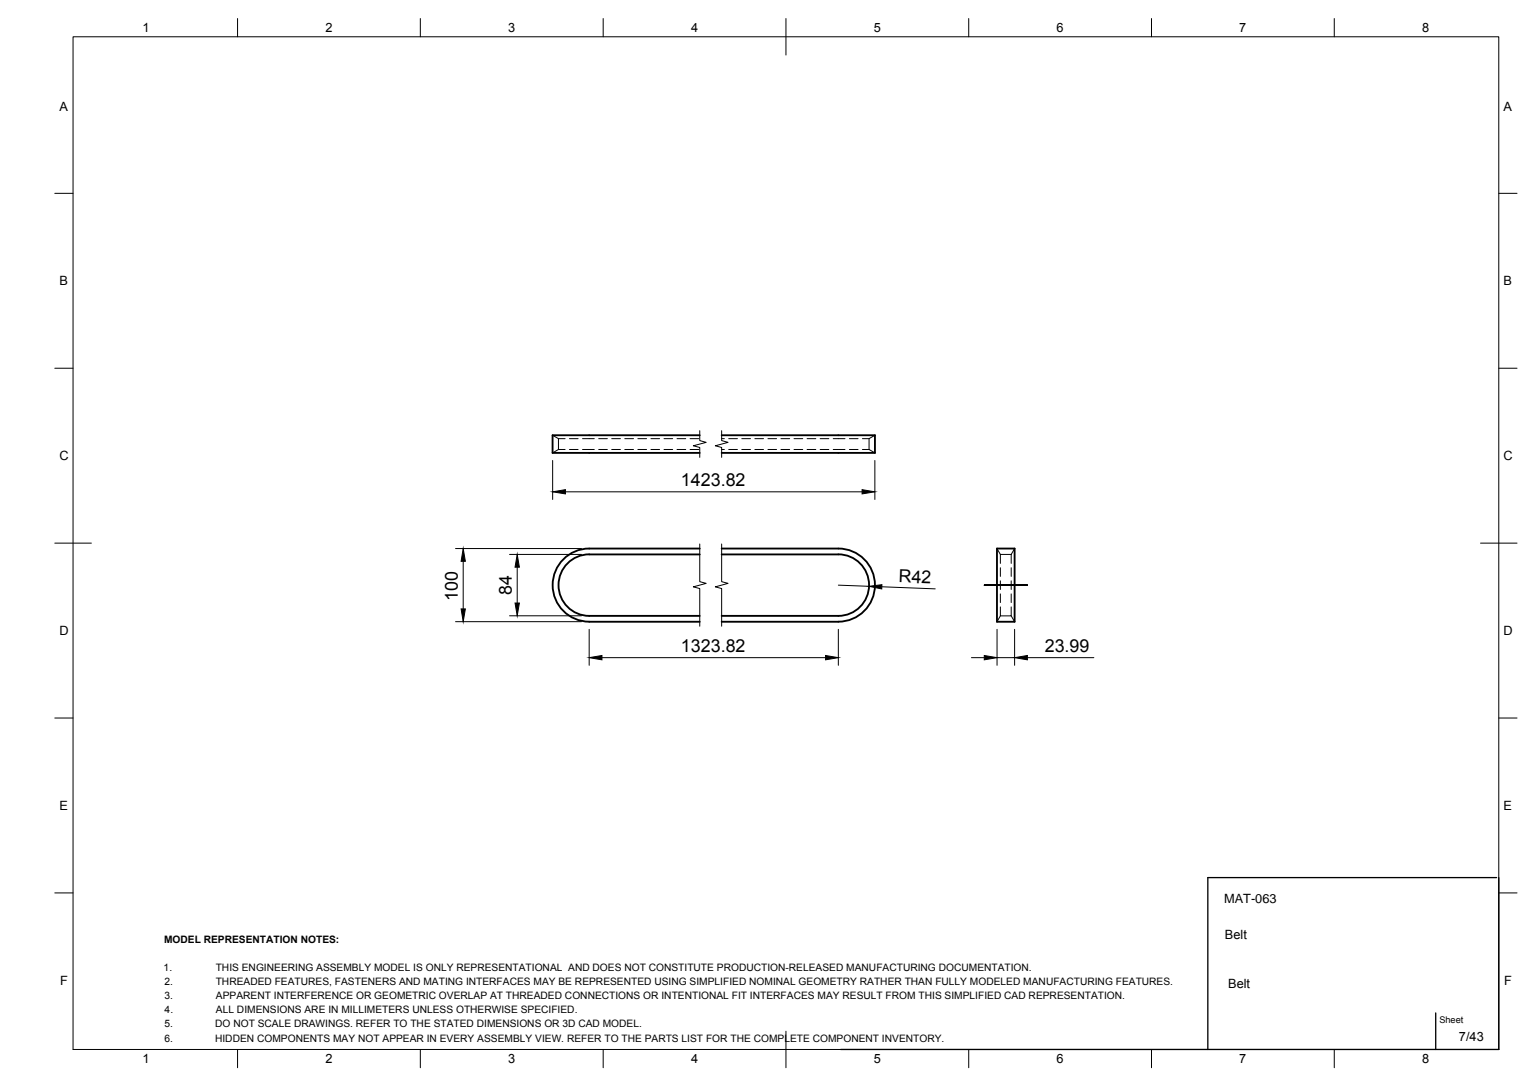
ISO-10303-21;
HEADER;
/* Generated by software containing ST-Developer
 * from STEP Tools, Inc. (www.steptools.com) 
 */

FILE_DESCRIPTION(
/* description */ (''),
/* implementation_level */ '2;1');

FILE_NAME(
/* name */ 'Belt.step',
/* time_stamp */ '2026-10-24T09:43:01-07:00',
/* author */ (''),
/* organization */ (''),
/* preprocessor_version */ 'ST-DEVELOPER v20.2',
/* originating_system */ 'Autodesk Translation Framework v15.15.0.0',
/* authorisation */ '');

FILE_SCHEMA (('AUTOMOTIVE_DESIGN { 1 0 10303 214 3 1 1 }'));
ENDSEC;

DATA;
#10=MECHANICAL_DESIGN_GEOMETRIC_PRESENTATION_REPRESENTATION('',(#277),#11112);
#211=SHAPE_REPRESENTATION_RELATIONSHIP('SRR','None',#11234,#244);
#244=ADVANCED_BREP_SHAPE_REPRESENTATION('',(#310),#11079);
#277=STYLED_ITEM('',(#11426),#310);
#310=MANIFOLD_SOLID_BREP('Belt',#6014);
#516=PLANE('',#6636);
#517=PLANE('',#6641);
#518=PLANE('',#6645);
#519=PLANE('',#6647);
#520=PLANE('',#6648);
#521=PLANE('',#6649);
#522=PLANE('',#6654);
#523=PLANE('',#6655);
#669=CONICAL_SURFACE('',#6637,1.,1.04719756558882);
#670=CONICAL_SURFACE('',#6639,1.,1.04719756558882);
#671=CONICAL_SURFACE('',#6650,1.,1.04719756558882);
#672=CONICAL_SURFACE('',#6652,1.,1.04719756558882);
#757=FACE_OUTER_BOUND('',#1165,.T.);
#758=FACE_OUTER_BOUND('',#1166,.T.);
#759=FACE_OUTER_BOUND('',#1167,.T.);
#760=FACE_OUTER_BOUND('',#1168,.T.);
#761=FACE_OUTER_BOUND('',#1169,.T.);
#762=FACE_OUTER_BOUND('',#1170,.T.);
#763=FACE_OUTER_BOUND('',#1171,.T.);
#764=FACE_OUTER_BOUND('',#1172,.T.);
#765=FACE_OUTER_BOUND('',#1173,.T.);
#766=FACE_OUTER_BOUND('',#1174,.T.);
#767=FACE_OUTER_BOUND('',#1175,.T.);
#768=FACE_OUTER_BOUND('',#1176,.T.);
#769=FACE_OUTER_BOUND('',#1177,.T.);
#770=FACE_OUTER_BOUND('',#1178,.T.);
#771=FACE_OUTER_BOUND('',#1179,.T.);
#772=FACE_OUTER_BOUND('',#1180,.T.);
#1165=EDGE_LOOP('',(#4313,#4314,#4315,#4316));
#1166=EDGE_LOOP('',(#4317,#4318,#4319,#4320));
#1167=EDGE_LOOP('',(#4321,#4322,#4323,#4324));
#1168=EDGE_LOOP('',(#4325,#4326,#4327,#4328));
#1169=EDGE_LOOP('',(#4329,#4330,#4331,#4332));
#1170=EDGE_LOOP('',(#4333,#4334,#4335,#4336));
#1171=EDGE_LOOP('',(#4337,#4338,#4339,#4340));
#1172=EDGE_LOOP('',(#4341,#4342,#4343,#4344));
#1173=EDGE_LOOP('',(#4345,#4346,#4347,#4348));
#1174=EDGE_LOOP('',(#4349,#4350,#4351,#4352));
#1175=EDGE_LOOP('',(#4353,#4354,#4355,#4356));
#1176=EDGE_LOOP('',(#4357,#4358,#4359,#4360));
#1177=EDGE_LOOP('',(#4361,#4362,#4363,#4364));
#1178=EDGE_LOOP('',(#4365,#4366,#4367,#4368));
#1179=EDGE_LOOP('',(#4369,#4370,#4371,#4372));
#1180=EDGE_LOOP('',(#4373,#4374,#4375,#4376));
#1602=LINE('',#9716,#1961);
#1603=LINE('',#9719,#1962);
#1604=LINE('',#9722,#1963);
#1605=LINE('',#9724,#1964);
#1606=LINE('',#9725,#1965);
#1607=LINE('',#9728,#1966);
#1608=LINE('',#9731,#1967);
#1609=LINE('',#9736,#1968);
#1610=LINE('',#9737,#1969);
#1611=LINE('',#9740,#1970);
#1612=LINE('',#9741,#1971);
#1613=LINE('',#9745,#1972);
#1614=LINE('',#9750,#1973);
#1615=LINE('',#9751,#1974);
#1616=LINE('',#9753,#1975);
#1617=LINE('',#9754,#1976);
#1618=LINE('',#9756,#1977);
#1619=LINE('',#9757,#1978);
#1620=LINE('',#9760,#1979);
#1621=LINE('',#9761,#1980);
#1622=LINE('',#9763,#1981);
#1623=LINE('',#9767,#1982);
#1624=LINE('',#9771,#1983);
#1625=LINE('',#9773,#1984);
#1961=VECTOR('',#7760,0.01);
#1962=VECTOR('',#7763,0.01);
#1963=VECTOR('',#7766,0.01);
#1964=VECTOR('',#7767,0.01);
#1965=VECTOR('',#7768,0.01);
#1966=VECTOR('',#7771,0.01);
#1967=VECTOR('',#7774,0.01);
#1968=VECTOR('',#7779,0.01);
#1969=VECTOR('',#7780,0.01);
#1970=VECTOR('',#7783,0.01);
#1971=VECTOR('',#7784,0.01);
#1972=VECTOR('',#7787,0.01);
#1973=VECTOR('',#7794,0.01);
#1974=VECTOR('',#7795,0.01);
#1975=VECTOR('',#7798,0.01);
#1976=VECTOR('',#7799,0.01);
#1977=VECTOR('',#7802,0.01);
#1978=VECTOR('',#7803,0.01);
#1979=VECTOR('',#7806,0.01);
#1980=VECTOR('',#7807,0.01);
#1981=VECTOR('',#7810,0.01);
#1982=VECTOR('',#7815,0.01);
#1983=VECTOR('',#7822,0.01);
#1984=VECTOR('',#7825,0.01);
#2412=CIRCLE('',#6634,0.042);
#2413=CIRCLE('',#6635,0.042);
#2414=CIRCLE('',#6638,0.05);
#2415=CIRCLE('',#6640,0.05);
#2416=CIRCLE('',#6643,0.0419999999999999);
#2417=CIRCLE('',#6644,0.0420000000000001);
#2418=CIRCLE('',#6651,0.05);
#2419=CIRCLE('',#6653,0.0500000000000661);
#2798=VERTEX_POINT('',#9712);
#2799=VERTEX_POINT('',#9713);
#2800=VERTEX_POINT('',#9715);
#2801=VERTEX_POINT('',#9717);
#2802=VERTEX_POINT('',#9721);
#2803=VERTEX_POINT('',#9723);
#2804=VERTEX_POINT('',#9727);
#2805=VERTEX_POINT('',#9729);
#2806=VERTEX_POINT('',#9733);
#2807=VERTEX_POINT('',#9734);
#2808=VERTEX_POINT('',#9739);
#2809=VERTEX_POINT('',#9743);
#2810=VERTEX_POINT('',#9744);
#2811=VERTEX_POINT('',#9749);
#2812=VERTEX_POINT('',#9759);
#2813=VERTEX_POINT('',#9765);
#3360=EDGE_CURVE('',#2798,#2799,#2412,.F.);
#3361=EDGE_CURVE('',#2800,#2798,#1602,.F.);
#3362=EDGE_CURVE('',#2801,#2800,#2413,.F.);
#3363=EDGE_CURVE('',#2799,#2801,#1603,.F.);
#3364=EDGE_CURVE('',#2802,#2801,#1604,.T.);
#3365=EDGE_CURVE('',#2803,#2802,#1605,.T.);
#3366=EDGE_CURVE('',#2799,#2803,#1606,.T.);
#3367=EDGE_CURVE('',#2804,#2800,#1607,.F.);
#3368=EDGE_CURVE('',#2805,#2804,#2414,.F.);
#3369=EDGE_CURVE('',#2801,#2805,#1608,.F.);
#3370=EDGE_CURVE('',#2806,#2807,#2415,.F.);
#3371=EDGE_CURVE('',#2798,#2806,#1609,.F.);
#3372=EDGE_CURVE('',#2807,#2799,#1610,.F.);
#3373=EDGE_CURVE('',#2808,#2805,#1611,.T.);
#3374=EDGE_CURVE('',#2802,#2808,#1612,.T.);
#3375=EDGE_CURVE('',#2809,#2810,#1613,.F.);
#3376=EDGE_CURVE('',#2803,#2809,#2416,.F.);
#3377=EDGE_CURVE('',#2810,#2802,#2417,.F.);
#3378=EDGE_CURVE('',#2807,#2811,#1614,.T.);
#3379=EDGE_CURVE('',#2811,#2803,#1615,.T.);
#3380=EDGE_CURVE('',#2804,#2806,#1616,.F.);
#3381=EDGE_CURVE('',#2807,#2805,#1617,.F.);
#3382=EDGE_CURVE('',#2800,#2810,#1618,.T.);
#3383=EDGE_CURVE('',#2809,#2798,#1619,.T.);
#3384=EDGE_CURVE('',#2812,#2806,#1620,.T.);
#3385=EDGE_CURVE('',#2809,#2812,#1621,.T.);
#3386=EDGE_CURVE('',#2808,#2811,#1622,.T.);
#3387=EDGE_CURVE('',#2813,#2808,#2418,.F.);
#3388=EDGE_CURVE('',#2810,#2813,#1623,.F.);
#3389=EDGE_CURVE('',#2811,#2812,#2419,.F.);
#3390=EDGE_CURVE('',#2804,#2813,#1624,.T.);
#3391=EDGE_CURVE('',#2812,#2813,#1625,.T.);
#4313=ORIENTED_EDGE('',*,*,#3360,.F.);
#4314=ORIENTED_EDGE('',*,*,#3361,.F.);
#4315=ORIENTED_EDGE('',*,*,#3362,.F.);
#4316=ORIENTED_EDGE('',*,*,#3363,.F.);
#4317=ORIENTED_EDGE('',*,*,#3363,.T.);
#4318=ORIENTED_EDGE('',*,*,#3364,.F.);
#4319=ORIENTED_EDGE('',*,*,#3365,.F.);
#4320=ORIENTED_EDGE('',*,*,#3366,.F.);
#4321=ORIENTED_EDGE('',*,*,#3362,.T.);
#4322=ORIENTED_EDGE('',*,*,#3367,.F.);
#4323=ORIENTED_EDGE('',*,*,#3368,.F.);
#4324=ORIENTED_EDGE('',*,*,#3369,.F.);
#4325=ORIENTED_EDGE('',*,*,#3370,.F.);
#4326=ORIENTED_EDGE('',*,*,#3371,.F.);
#4327=ORIENTED_EDGE('',*,*,#3360,.T.);
#4328=ORIENTED_EDGE('',*,*,#3372,.F.);
#4329=ORIENTED_EDGE('',*,*,#3369,.T.);
#4330=ORIENTED_EDGE('',*,*,#3373,.F.);
#4331=ORIENTED_EDGE('',*,*,#3374,.F.);
#4332=ORIENTED_EDGE('',*,*,#3364,.T.);
#4333=ORIENTED_EDGE('',*,*,#3375,.F.);
#4334=ORIENTED_EDGE('',*,*,#3376,.F.);
#4335=ORIENTED_EDGE('',*,*,#3365,.T.);
#4336=ORIENTED_EDGE('',*,*,#3377,.F.);
#4337=ORIENTED_EDGE('',*,*,#3378,.F.);
#4338=ORIENTED_EDGE('',*,*,#3372,.T.);
#4339=ORIENTED_EDGE('',*,*,#3366,.T.);
#4340=ORIENTED_EDGE('',*,*,#3379,.F.);
#4341=ORIENTED_EDGE('',*,*,#3368,.T.);
#4342=ORIENTED_EDGE('',*,*,#3380,.T.);
#4343=ORIENTED_EDGE('',*,*,#3370,.T.);
#4344=ORIENTED_EDGE('',*,*,#3381,.T.);
#4345=ORIENTED_EDGE('',*,*,#3382,.F.);
#4346=ORIENTED_EDGE('',*,*,#3361,.T.);
#4347=ORIENTED_EDGE('',*,*,#3383,.F.);
#4348=ORIENTED_EDGE('',*,*,#3375,.T.);
#4349=ORIENTED_EDGE('',*,*,#3371,.T.);
#4350=ORIENTED_EDGE('',*,*,#3384,.F.);
#4351=ORIENTED_EDGE('',*,*,#3385,.F.);
#4352=ORIENTED_EDGE('',*,*,#3383,.T.);
#4353=ORIENTED_EDGE('',*,*,#3381,.F.);
#4354=ORIENTED_EDGE('',*,*,#3378,.T.);
#4355=ORIENTED_EDGE('',*,*,#3386,.F.);
#4356=ORIENTED_EDGE('',*,*,#3373,.T.);
#4357=ORIENTED_EDGE('',*,*,#3377,.T.);
#4358=ORIENTED_EDGE('',*,*,#3374,.T.);
#4359=ORIENTED_EDGE('',*,*,#3387,.F.);
#4360=ORIENTED_EDGE('',*,*,#3388,.F.);
#4361=ORIENTED_EDGE('',*,*,#3376,.T.);
#4362=ORIENTED_EDGE('',*,*,#3385,.T.);
#4363=ORIENTED_EDGE('',*,*,#3389,.F.);
#4364=ORIENTED_EDGE('',*,*,#3379,.T.);
#4365=ORIENTED_EDGE('',*,*,#3367,.T.);
#4366=ORIENTED_EDGE('',*,*,#3382,.T.);
#4367=ORIENTED_EDGE('',*,*,#3388,.T.);
#4368=ORIENTED_EDGE('',*,*,#3390,.F.);
#4369=ORIENTED_EDGE('',*,*,#3380,.F.);
#4370=ORIENTED_EDGE('',*,*,#3390,.T.);
#4371=ORIENTED_EDGE('',*,*,#3391,.F.);
#4372=ORIENTED_EDGE('',*,*,#3384,.T.);
#4373=ORIENTED_EDGE('',*,*,#3391,.T.);
#4374=ORIENTED_EDGE('',*,*,#3387,.T.);
#4375=ORIENTED_EDGE('',*,*,#3386,.T.);
#4376=ORIENTED_EDGE('',*,*,#3389,.T.);
#5539=CYLINDRICAL_SURFACE('',#6633,0.042);
#5540=CYLINDRICAL_SURFACE('',#6642,0.042);
#5541=CYLINDRICAL_SURFACE('',#6646,0.05);
#5542=CYLINDRICAL_SURFACE('',#6656,0.05);
#5730=ADVANCED_FACE('',(#757),#5539,.F.);
#5731=ADVANCED_FACE('',(#758),#516,.F.);
#5732=ADVANCED_FACE('',(#759),#669,.F.);
#5733=ADVANCED_FACE('',(#760),#670,.F.);
#5734=ADVANCED_FACE('',(#761),#517,.F.);
#5735=ADVANCED_FACE('',(#762),#5540,.F.);
#5736=ADVANCED_FACE('',(#763),#518,.F.);
#5737=ADVANCED_FACE('',(#764),#5541,.T.);
#5738=ADVANCED_FACE('',(#765),#519,.F.);
#5739=ADVANCED_FACE('',(#766),#520,.F.);
#5740=ADVANCED_FACE('',(#767),#521,.F.);
#5741=ADVANCED_FACE('',(#768),#671,.F.);
#5742=ADVANCED_FACE('',(#769),#672,.F.);
#5743=ADVANCED_FACE('',(#770),#522,.F.);
#5744=ADVANCED_FACE('',(#771),#523,.F.);
#5745=ADVANCED_FACE('',(#772),#5542,.T.);
#6014=CLOSED_SHELL('',(#5730,#5731,#5732,#5733,#5734,#5735,#5736,#5737,
#5738,#5739,#5740,#5741,#5742,#5743,#5744,#5745));
#6632=AXIS2_PLACEMENT_3D('',#9710,#7754,#7755);
#6633=AXIS2_PLACEMENT_3D('',#9711,#7756,#7757);
#6634=AXIS2_PLACEMENT_3D('',#9714,#7758,#7759);
#6635=AXIS2_PLACEMENT_3D('',#9718,#7761,#7762);
#6636=AXIS2_PLACEMENT_3D('',#9720,#7764,#7765);
#6637=AXIS2_PLACEMENT_3D('',#9726,#7769,#7770);
#6638=AXIS2_PLACEMENT_3D('',#9730,#7772,#7773);
#6639=AXIS2_PLACEMENT_3D('',#9732,#7775,#7776);
#6640=AXIS2_PLACEMENT_3D('',#9735,#7777,#7778);
#6641=AXIS2_PLACEMENT_3D('',#9738,#7781,#7782);
#6642=AXIS2_PLACEMENT_3D('',#9742,#7785,#7786);
#6643=AXIS2_PLACEMENT_3D('',#9746,#7788,#7789);
#6644=AXIS2_PLACEMENT_3D('',#9747,#7790,#7791);
#6645=AXIS2_PLACEMENT_3D('',#9748,#7792,#7793);
#6646=AXIS2_PLACEMENT_3D('',#9752,#7796,#7797);
#6647=AXIS2_PLACEMENT_3D('',#9755,#7800,#7801);
#6648=AXIS2_PLACEMENT_3D('',#9758,#7804,#7805);
#6649=AXIS2_PLACEMENT_3D('',#9762,#7808,#7809);
#6650=AXIS2_PLACEMENT_3D('',#9764,#7811,#7812);
#6651=AXIS2_PLACEMENT_3D('',#9766,#7813,#7814);
#6652=AXIS2_PLACEMENT_3D('',#9768,#7816,#7817);
#6653=AXIS2_PLACEMENT_3D('',#9769,#7818,#7819);
#6654=AXIS2_PLACEMENT_3D('',#9770,#7820,#7821);
#6655=AXIS2_PLACEMENT_3D('',#9772,#7823,#7824);
#6656=AXIS2_PLACEMENT_3D('',#9774,#7826,#7827);
#7754=DIRECTION('axis',(0.,0.,1.));
#7755=DIRECTION('refdir',(1.,0.,0.));
#7756=DIRECTION('center_axis',(0.,0.,1.));
#7757=DIRECTION('ref_axis',(1.,0.,0.));
#7758=DIRECTION('center_axis',(0.,0.,-1.));
#7759=DIRECTION('ref_axis',(1.,2.500007018071E-10,0.));
#7760=DIRECTION('',(0.,0.,1.));
#7761=DIRECTION('center_axis',(-2.35325480076137E-17,4.40779226798152E-17,
1.));
#7762=DIRECTION('ref_axis',(1.,-4.29586600835191E-10,2.64338815386942E-17));
#7763=DIRECTION('',(0.,0.,-1.));
#7764=DIRECTION('center_axis',(0.556379847069157,0.830928074971175,-7.35361873603602E-16));
#7765=DIRECTION('ref_axis',(-0.830928074971175,0.556379847069157,7.16694797445736E-33));
#7766=DIRECTION('',(0.830928075153644,-0.556379846796646,-5.68042456784337E-10));
#7767=DIRECTION('',(0.,0.,1.));
#7768=DIRECTION('',(-0.830928075153644,0.556379846796646,-5.6804240310886E-10));
#7769=DIRECTION('center_axis',(0.,0.,1.));
#7770=DIRECTION('ref_axis',(1.,0.,0.));
#7771=DIRECTION('',(-0.481839085130227,-0.719604828016666,0.499999987535971));
#7772=DIRECTION('center_axis',(0.,0.,1.));
#7773=DIRECTION('ref_axis',(1.,-4.29586566999823E-10,0.));
#7774=DIRECTION('',(-0.481839085425413,-0.719604827819009,-0.499999987535975));
#7775=DIRECTION('center_axis',(0.,0.,-1.));
#7776=DIRECTION('ref_axis',(0.830928075019912,-0.556379846996369,0.));
#7777=DIRECTION('center_axis',(-3.95346806367293E-17,7.40509100908303E-17,
-1.));
#7778=DIRECTION('ref_axis',(-0.556379846372783,-0.830928075437459,-4.44089209850062E-17));
#7779=DIRECTION('',(0.481839085296186,0.719604827905541,0.499999987535972));
#7780=DIRECTION('',(0.481839085720606,0.719604827621357,-0.499999987535967));
#7781=DIRECTION('center_axis',(0.278189923027056,0.41546403790653,-0.866025403745526));
#7782=DIRECTION('ref_axis',(-1.21325454929337E-16,0.901615702162283,0.432538004820864));
#7783=DIRECTION('',(0.8309280753204,-0.556379846547604,-3.68626283987023E-10));
#7784=DIRECTION('',(0.481839111062359,0.719604801945691,0.500000000067339));
#7785=DIRECTION('center_axis',(0.,0.,1.));
#7786=DIRECTION('ref_axis',(-0.830928076007245,0.556379845521832,0.));
#7787=DIRECTION('',(0.,0.,-1.));
#7788=DIRECTION('center_axis',(1.97868596828159E-16,1.05639103603771E-16,
-1.));
#7789=DIRECTION('ref_axis',(-1.,-4.10213239038492E-10,-1.8503717077086E-16));
#7790=DIRECTION('center_axis',(0.,0.,1.));
#7791=DIRECTION('ref_axis',(-0.556379848848799,-0.830928073779547,0.));
#7792=DIRECTION('center_axis',(0.278189923027056,0.41546403790653,0.866025403745527));
#7793=DIRECTION('ref_axis',(7.03710115468502E-19,-0.901615702162283,0.432538004820864));
#7794=DIRECTION('',(-0.8309280753204,0.556379846547604,-3.68626057553233E-10));
#7795=DIRECTION('',(-0.481839111062391,-0.719604801945631,0.500000000067394));
#7796=DIRECTION('center_axis',(0.,0.,1.));
#7797=DIRECTION('ref_axis',(1.,0.,0.));
#7798=DIRECTION('',(0.,0.,1.));
#7799=DIRECTION('',(0.,0.,-1.));
#7800=DIRECTION('center_axis',(-0.556379846547605,-0.8309280753204,1.01878114391287E-15));
#7801=DIRECTION('ref_axis',(0.8309280753204,-0.556379846547605,8.47369377023234E-32));
#7802=DIRECTION('',(-0.830928075329978,0.5563798465333,-2.98215105322737E-11));
#7803=DIRECTION('',(0.830928075329979,-0.556379846533299,-2.98209335407452E-11));
#7804=DIRECTION('center_axis',(-0.278189923198529,-0.415464037609672,0.866025403832859));
#7805=DIRECTION('ref_axis',(-8.10651120153385E-17,-0.90161570229982,-0.43253800453417));
#7806=DIRECTION('',(0.830928074971174,-0.556379847069157,-3.67583016147327E-10));
#7807=DIRECTION('',(-0.481839110724413,-0.719604802277015,-0.499999999916165));
#7808=DIRECTION('center_axis',(-0.556379846547604,-0.8309280753204,-1.1124685724156E-15));
#7809=DIRECTION('ref_axis',(0.8309280753204,-0.556379846547604,-7.86302266460809E-32));
#7810=DIRECTION('',(0.,0.,-1.));
#7811=DIRECTION('center_axis',(0.,0.,1.));
#7812=DIRECTION('ref_axis',(-0.830928074495347,0.556379847779784,0.));
#7813=DIRECTION('center_axis',(0.,0.,1.));
#7814=DIRECTION('ref_axis',(-0.556379846596556,-0.830928075287622,0.));
#7815=DIRECTION('',(0.481839085129936,0.7196048280168,-0.499999987536058));
#7816=DIRECTION('center_axis',(0.,0.,-1.));
#7817=DIRECTION('ref_axis',(-1.,0.,0.));
#7818=DIRECTION('center_axis',(-1.88631312013914E-13,-1.0754841012286E-13,
-1.));
#7819=DIRECTION('ref_axis',(-1.,-4.29767510467514E-10,1.88649096344057E-13));
#7820=DIRECTION('center_axis',(-0.278189923198529,-0.415464037609672,-0.866025403832859));
#7821=DIRECTION('ref_axis',(8.10651120153385E-17,0.90161570229982,-0.43253800453417));
#7822=DIRECTION('',(-0.830928074971174,0.556379847069157,-3.67583167123921E-10));
#7823=DIRECTION('center_axis',(0.556379847069157,0.830928074971175,2.1611143699565E-16));
#7824=DIRECTION('ref_axis',(-0.830928074971175,0.556379847069157,8.67438128407877E-33));
#7825=DIRECTION('',(0.,0.,1.));
#7826=DIRECTION('center_axis',(0.,0.,1.));
#7827=DIRECTION('ref_axis',(-0.830928075876665,0.556379845716848,0.));
#9710=CARTESIAN_POINT('',(0.,0.,0.));
#9711=CARTESIAN_POINT('Origin',(0.,0.,-7.87263173541793E-35));
#9712=CARTESIAN_POINT('',(-0.0233679536357646,-0.034898979153486,-0.00737500014596191));
#9713=CARTESIAN_POINT('',(0.0233679535551443,0.0348989792127245,-0.00737499998943404));
#9714=CARTESIAN_POINT('Origin',(4.44089209850063E-17,-3.10862446895044E-17,
-0.007375));
#9715=CARTESIAN_POINT('',(-0.0233679536079189,-0.0348989791421631,0.00737500011314446));
#9716=CARTESIAN_POINT('',(-0.0233679535483332,-0.0348989791679204,-0.00737499975));
#9717=CARTESIAN_POINT('',(0.0233679535131933,0.0348989792427655,0.00737499998724119));
#9718=CARTESIAN_POINT('Origin',(1.77635683940025E-17,8.88178419700125E-18,
0.007375));
#9719=CARTESIAN_POINT('',(0.023367953562649,0.0348989791583347,0.00737499975));
#9720=CARTESIAN_POINT('Origin',(-0.526632046,0.40317263,-3.19189119579732E-18));
#9721=CARTESIAN_POINT('',(-1.0766320462855,0.771446280610377,0.00737500043869704));
#9722=CARTESIAN_POINT('',(-1.07663204595213,0.771446280476663,0.00737500070705611));
#9723=CARTESIAN_POINT('',(-1.07663204628435,0.771446280609598,-0.00737500043868999));
#9724=CARTESIAN_POINT('',(-1.076632046,0.771446281,-0.00737499999631251));
#9725=CARTESIAN_POINT('',(0.0233679534964875,0.034898979368365,-0.00737499995506969));
#9726=CARTESIAN_POINT('Origin',(0.,0.,0.560476539500209));
#9727=CARTESIAN_POINT('',(-0.0278189923670676,-0.0415464037720794,0.011993802156313));
#9728=CARTESIAN_POINT('',(-0.0233679536799733,-0.034898979364519,0.00737500013681456));
#9729=CARTESIAN_POINT('',(0.0278189923276001,0.0415464037677099,0.0119938019829276));
#9730=CARTESIAN_POINT('Origin',(1.33226762955019E-17,8.88178419700125E-18,
0.0119938020001596));
#9731=CARTESIAN_POINT('',(0.0278189922159758,0.0415464035799445,0.0119938018751596));
#9732=CARTESIAN_POINT('Origin',(0.,0.,-0.560476539500202));
#9733=CARTESIAN_POINT('',(-0.0278189923461909,-0.0415464037862849,-0.0119938021566348));
#9734=CARTESIAN_POINT('',(0.0278189923407346,0.0415464037588361,-0.0119938019828069));
#9735=CARTESIAN_POINT('Origin',(2.66453525910038E-17,1.32781373427172E-17,
-0.0119938020001543));
#9736=CARTESIAN_POINT('',(-0.0278189922085164,-0.041546403584943,-0.0119938018751542));
#9737=CARTESIAN_POINT('',(0.023367953697375,0.0348989793285763,-0.00737500012515425));
#9738=CARTESIAN_POINT('Origin',(-0.524406527000001,0.406496342,0.00968440124999999));
#9739=CARTESIAN_POINT('',(-1.0721810077487,0.778093704786141,0.0119938023047236));
#9740=CARTESIAN_POINT('',(-1.07218100730026,0.778093704531458,0.0119938024396044));
#9741=CARTESIAN_POINT('',(-1.07663204644624,0.77144628044497,0.00737500053312992));
#9742=CARTESIAN_POINT('Origin',(-1.1,0.736547301,-1.65083181236565E-33));
#9743=CARTESIAN_POINT('',(-1.12336795372113,0.701648321968335,-0.00737500014124816));
#9744=CARTESIAN_POINT('',(-1.12336795361188,0.701648321848912,0.00737500010599789));
#9745=CARTESIAN_POINT('',(-1.12336795354833,0.70164832183208,0.00737499975));
#9746=CARTESIAN_POINT('Origin',(-1.1,0.736547301,-0.00737499999999999));
#9747=CARTESIAN_POINT('Origin',(-1.1,0.736547301,0.007375));
#9748=CARTESIAN_POINT('Origin',(-0.524406527000001,0.406496342,-0.00968440125000005));
#9749=CARTESIAN_POINT('',(-1.07218100774996,0.778093704787018,-0.0119938023047757));
#9750=CARTESIAN_POINT('',(0.0278189920263111,0.0415464039823829,-0.0119938019516094));
#9751=CARTESIAN_POINT('',(-1.07218100773738,0.778093704356822,-0.011993802335713));
#9752=CARTESIAN_POINT('Origin',(0.,0.,-2.35699650765267E-35));
#9753=CARTESIAN_POINT('',(-0.0278189923194442,-0.0415464037713338,-0.01199380175));
#9754=CARTESIAN_POINT('',(0.0278189923364869,0.0415464037599223,0.01199380175));
#9755=CARTESIAN_POINT('Origin',(-0.573367954,0.333374671499999,-3.19189119579732E-18));
#9756=CARTESIAN_POINT('',(-0.0233679541909832,-0.0348989786903893,0.00737500026154926));
#9757=CARTESIAN_POINT('',(-1.1233679536435,0.701648321915596,-0.00737500022207161));
#9758=CARTESIAN_POINT('Origin',(-0.575593473000001,0.33005095925,-0.00968440124999998));
#9759=CARTESIAN_POINT('',(-1.12781899223605,0.69500089782109,-0.011993801966612));
#9760=CARTESIAN_POINT('',(-1.12781899190905,0.695000897939099,-0.0119938018658674));
#9761=CARTESIAN_POINT('',(-1.12336795377236,0.701648322288803,-0.00737500008442041));
#9762=CARTESIAN_POINT('Origin',(-0.522181008,0.4098200545,-6.67868538251071E-19));
#9763=CARTESIAN_POINT('',(-1.072181008,0.778093705,0.0119938018623003));
#9764=CARTESIAN_POINT('Origin',(-1.1,0.736547301,0.560476539499858));
#9765=CARTESIAN_POINT('',(-1.12781899207711,0.695000897561786,0.0119938019516492));
#9766=CARTESIAN_POINT('Origin',(-1.1,0.736547301,0.0119938019998959));
#9767=CARTESIAN_POINT('',(-1.1278189920545,0.695000897624348,0.0119938017249309));
#9768=CARTESIAN_POINT('Origin',(-1.1,0.736547301,-0.560476539499883));
#9769=CARTESIAN_POINT('Origin',(-1.09999999999998,0.736547301000009,-0.011993801999925));
#9770=CARTESIAN_POINT('Origin',(-0.575593473000001,0.33005095925,0.00968440125000007));
#9771=CARTESIAN_POINT('',(-0.0278189926997751,-0.0415464035314387,0.0119938023524818));
#9772=CARTESIAN_POINT('Origin',(-0.577818992,0.326727247,-6.67868538251071E-19));
#9773=CARTESIAN_POINT('',(-1.127818992,0.695000898,-0.0119938018016607));
#9774=CARTESIAN_POINT('Origin',(-1.1,0.736547301,-1.37226748941978E-34));
#11040=UNCERTAINTY_MEASURE_WITH_UNIT(LENGTH_MEASURE(1.E-5),#11113,
'DISTANCE_ACCURACY_VALUE',
'Maximum model space distance between geometric entities at asserted c
onnectivities');
#11073=UNCERTAINTY_MEASURE_WITH_UNIT(LENGTH_MEASURE(1.E-5),#11113,
'DISTANCE_ACCURACY_VALUE',
'Maximum model space distance between geometric entities at asserted c
onnectivities');
#11079=(
GEOMETRIC_REPRESENTATION_CONTEXT(3)
GLOBAL_UNCERTAINTY_ASSIGNED_CONTEXT((#11040))
GLOBAL_UNIT_ASSIGNED_CONTEXT((#11113,#11114,#11115))
REPRESENTATION_CONTEXT('','3D')
);
#11112=(
GEOMETRIC_REPRESENTATION_CONTEXT(3)
GLOBAL_UNCERTAINTY_ASSIGNED_CONTEXT((#11073))
GLOBAL_UNIT_ASSIGNED_CONTEXT((#11113,#11114,#11115))
REPRESENTATION_CONTEXT('','3D')
);
#11113=(
LENGTH_UNIT()
NAMED_UNIT(*)
SI_UNIT($,.METRE.)
);
#11114=(
NAMED_UNIT(*)
PLANE_ANGLE_UNIT()
SI_UNIT($,.RADIAN.)
);
#11115=(
NAMED_UNIT(*)
SI_UNIT($,.STERADIAN.)
SOLID_ANGLE_UNIT()
);
#11121=SHAPE_DEFINITION_REPRESENTATION(#11159,#11234);
#11159=PRODUCT_DEFINITION_SHAPE('',$,#11273);
#11234=SHAPE_REPRESENTATION('',(#6632),#11079);
#11267=PRODUCT_DEFINITION_CONTEXT('part definition',#11383,'design');
#11273=PRODUCT_DEFINITION('Belt','Belt',#11311,#11267);
#11311=PRODUCT_DEFINITION_FORMATION('',$,#11390);
#11383=APPLICATION_CONTEXT(
'Core Data for Automotive Mechanical Design Process');
#11384=PRODUCT_CONTEXT('part definition',#11383,'mechanical');
#11390=PRODUCT('Belt','Belt','Belt1-13__ DE    13309',(#11384));
#11426=PRESENTATION_STYLE_ASSIGNMENT((#11430));
#11430=SURFACE_STYLE_USAGE(.BOTH.,#11434);
#11434=SURFACE_SIDE_STYLE('',(#11438));
#11438=SURFACE_STYLE_FILL_AREA(#11442);
#11442=FILL_AREA_STYLE('Opaque(202,209,238)',(#11446));
#11446=FILL_AREA_STYLE_COLOUR('Opaque(202,209,238)',#11450);
#11450=COLOUR_RGB('Opaque(202,209,238)',0.792156862745098,0.819607843137255,
0.933333333333333);
ENDSEC;
END-ISO-10303-21;
